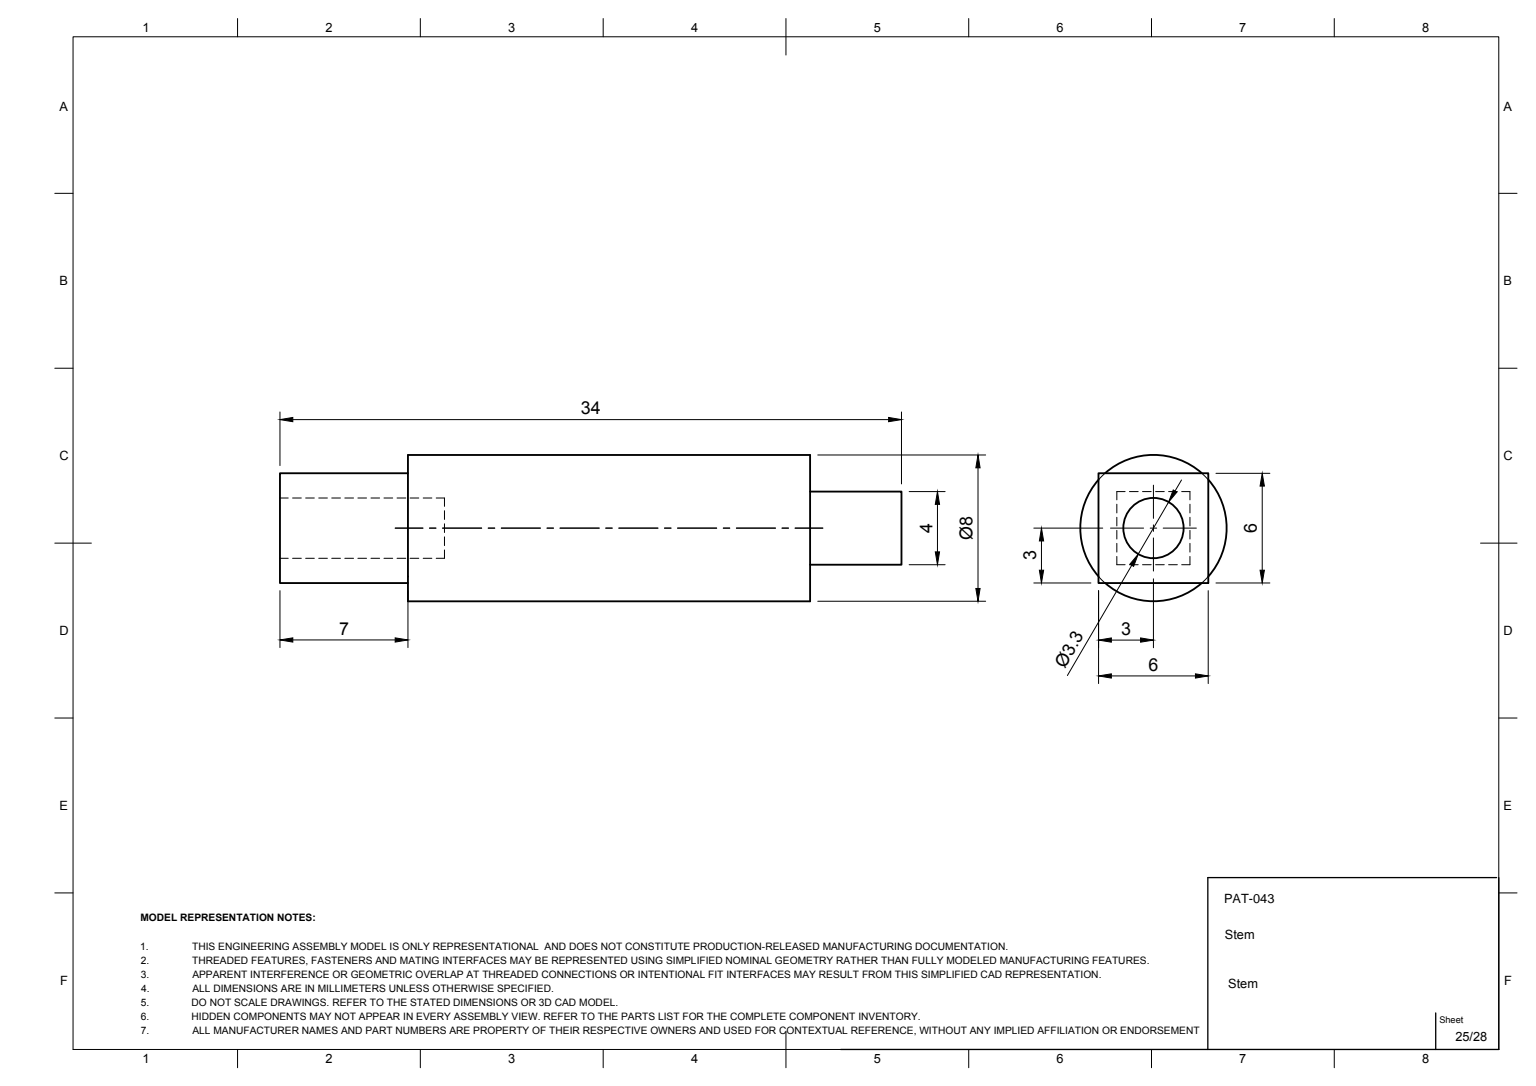
ISO-10303-21;
HEADER;
/* Generated by software containing ST-Developer
 * from STEP Tools, Inc. (www.steptools.com) 
 */

FILE_DESCRIPTION(
/* description */ ('Four-valve pipe header'),
/* implementation_level */ '2;1');

FILE_NAME(
/* name */ 'Stem.step',
/* time_stamp */ '2026-10-29T16:56:19-07:00',
/* author */ (''),
/* organization */ (''),
/* preprocessor_version */ 'ST-DEVELOPER v20.2',
/* originating_system */ 'Autodesk Translation Framework v15.17.0.0',
/* authorisation */ '');

FILE_SCHEMA (('AUTOMOTIVE_DESIGN { 1 0 10303 214 3 1 1 }'));
ENDSEC;

DATA;
#10=MECHANICAL_DESIGN_GEOMETRIC_PRESENTATION_REPRESENTATION('',(#354),#10119);
#302=SHAPE_REPRESENTATION_RELATIONSHIP('SRR','None',#10265,#328);
#328=ADVANCED_BREP_SHAPE_REPRESENTATION('',(#378),#10114);
#354=STYLED_ITEM('',(#10463),#378);
#378=MANIFOLD_SOLID_BREP('Body1',#5602);
#528=FACE_BOUND('',#1466,.T.);
#529=FACE_BOUND('',#1478,.T.);
#698=PLANE('',#6431);
#699=PLANE('',#6432);
#700=PLANE('',#6434);
#701=PLANE('',#6436);
#702=PLANE('',#6438);
#703=PLANE('',#6440);
#704=PLANE('',#6441);
#705=PLANE('',#6442);
#706=PLANE('',#6443);
#707=PLANE('',#6444);
#708=PLANE('',#6445);
#709=PLANE('',#6447);
#710=PLANE('',#6450);
#711=PLANE('',#6452);
#712=PLANE('',#6454);
#713=PLANE('',#6455);
#714=PLANE('',#6456);
#715=PLANE('',#6457);
#716=PLANE('',#6458);
#717=PLANE('',#6461);
#1021=FACE_OUTER_BOUND('',#1455,.T.);
#1022=FACE_OUTER_BOUND('',#1456,.T.);
#1023=FACE_OUTER_BOUND('',#1457,.T.);
#1024=FACE_OUTER_BOUND('',#1458,.T.);
#1025=FACE_OUTER_BOUND('',#1459,.T.);
#1026=FACE_OUTER_BOUND('',#1460,.T.);
#1027=FACE_OUTER_BOUND('',#1461,.T.);
#1028=FACE_OUTER_BOUND('',#1462,.T.);
#1029=FACE_OUTER_BOUND('',#1463,.T.);
#1030=FACE_OUTER_BOUND('',#1464,.T.);
#1031=FACE_OUTER_BOUND('',#1465,.T.);
#1032=FACE_OUTER_BOUND('',#1467,.T.);
#1033=FACE_OUTER_BOUND('',#1468,.T.);
#1034=FACE_OUTER_BOUND('',#1469,.T.);
#1035=FACE_OUTER_BOUND('',#1470,.T.);
#1036=FACE_OUTER_BOUND('',#1471,.T.);
#1037=FACE_OUTER_BOUND('',#1472,.T.);
#1038=FACE_OUTER_BOUND('',#1473,.T.);
#1039=FACE_OUTER_BOUND('',#1474,.T.);
#1040=FACE_OUTER_BOUND('',#1475,.T.);
#1041=FACE_OUTER_BOUND('',#1476,.T.);
#1042=FACE_OUTER_BOUND('',#1477,.T.);
#1455=EDGE_LOOP('',(#4913,#4914,#4915,#4916));
#1456=EDGE_LOOP('',(#4917));
#1457=EDGE_LOOP('',(#4918,#4919,#4920));
#1458=EDGE_LOOP('',(#4921,#4922,#4923));
#1459=EDGE_LOOP('',(#4924,#4925,#4926));
#1460=EDGE_LOOP('',(#4927,#4928,#4929));
#1461=EDGE_LOOP('',(#4930,#4931,#4932,#4933,#4934,#4935));
#1462=EDGE_LOOP('',(#4936,#4937,#4938,#4939,#4940,#4941));
#1463=EDGE_LOOP('',(#4942,#4943,#4944,#4945,#4946,#4947));
#1464=EDGE_LOOP('',(#4948,#4949,#4950,#4951,#4952,#4953));
#1465=EDGE_LOOP('',(#4954,#4955,#4956,#4957));
#1466=EDGE_LOOP('',(#4958));
#1467=EDGE_LOOP('',(#4959,#4960));
#1468=EDGE_LOOP('',(#4961,#4962,#4963));
#1469=EDGE_LOOP('',(#4964,#4965));
#1470=EDGE_LOOP('',(#4966,#4967));
#1471=EDGE_LOOP('',(#4968,#4969,#4970,#4971));
#1472=EDGE_LOOP('',(#4972,#4973,#4974,#4975));
#1473=EDGE_LOOP('',(#4976,#4977,#4978,#4979));
#1474=EDGE_LOOP('',(#4980,#4981,#4982,#4983));
#1475=EDGE_LOOP('',(#4984,#4985,#4986,#4987));
#1476=EDGE_LOOP('',(#4988,#4989,#4990,#4991,#4992,#4993,#4994,#4995,#4996,
#4997,#4998,#4999));
#1477=EDGE_LOOP('',(#5000));
#1478=EDGE_LOOP('',(#5001,#5002,#5003,#5004));
#1843=LINE('',#9751,#2261);
#1844=LINE('',#9759,#2262);
#1845=LINE('',#9760,#2263);
#1846=LINE('',#9766,#2264);
#1847=LINE('',#9767,#2265);
#1848=LINE('',#9773,#2266);
#1849=LINE('',#9774,#2267);
#1850=LINE('',#9780,#2268);
#1851=LINE('',#9781,#2269);
#1852=LINE('',#9783,#2270);
#1853=LINE('',#9785,#2271);
#1854=LINE('',#9787,#2272);
#1855=LINE('',#9788,#2273);
#1856=LINE('',#9790,#2274);
#1857=LINE('',#9792,#2275);
#1858=LINE('',#9793,#2276);
#1859=LINE('',#9795,#2277);
#1860=LINE('',#9797,#2278);
#1861=LINE('',#9798,#2279);
#1862=LINE('',#9800,#2280);
#1863=LINE('',#9801,#2281);
#1864=LINE('',#9816,#2282);
#1865=LINE('',#9818,#2283);
#1866=LINE('',#9820,#2284);
#1867=LINE('',#9821,#2285);
#1868=LINE('',#9824,#2286);
#1869=LINE('',#9826,#2287);
#1870=LINE('',#9827,#2288);
#1871=LINE('',#9830,#2289);
#1872=LINE('',#9832,#2290);
#1873=LINE('',#9833,#2291);
#1874=LINE('',#9835,#2292);
#1875=LINE('',#9836,#2293);
#1876=LINE('',#9840,#2294);
#2261=VECTOR('',#7962,0.165);
#2262=VECTOR('',#7971,1.);
#2263=VECTOR('',#7972,1.);
#2264=VECTOR('',#7977,1.);
#2265=VECTOR('',#7978,1.);
#2266=VECTOR('',#7983,1.);
#2267=VECTOR('',#7984,1.);
#2268=VECTOR('',#7989,1.);
#2269=VECTOR('',#7990,1.);
#2270=VECTOR('',#7993,1.);
#2271=VECTOR('',#7994,1.);
#2272=VECTOR('',#7995,1.);
#2273=VECTOR('',#7996,1.);
#2274=VECTOR('',#7999,1.);
#2275=VECTOR('',#8000,1.);
#2276=VECTOR('',#8001,1.);
#2277=VECTOR('',#8004,1.);
#2278=VECTOR('',#8005,1.);
#2279=VECTOR('',#8006,1.);
#2280=VECTOR('',#8009,1.);
#2281=VECTOR('',#8010,1.);
#2282=VECTOR('',#8033,1.);
#2283=VECTOR('',#8034,1.);
#2284=VECTOR('',#8035,1.);
#2285=VECTOR('',#8036,1.);
#2286=VECTOR('',#8039,1.);
#2287=VECTOR('',#8040,1.);
#2288=VECTOR('',#8041,1.);
#2289=VECTOR('',#8044,1.);
#2290=VECTOR('',#8045,1.);
#2291=VECTOR('',#8046,1.);
#2292=VECTOR('',#8049,1.);
#2293=VECTOR('',#8050,1.);
#2294=VECTOR('',#8055,0.4);
#2557=CIRCLE('',#6429,0.165);
#2558=CIRCLE('',#6430,0.165);
#2559=CIRCLE('',#6433,0.4);
#2560=CIRCLE('',#6435,0.4);
#2561=CIRCLE('',#6437,0.4);
#2562=CIRCLE('',#6439,0.4);
#2563=CIRCLE('',#6446,0.4);
#2564=CIRCLE('',#6448,0.4);
#2565=CIRCLE('',#6449,0.4);
#2566=CIRCLE('',#6451,0.4);
#2567=CIRCLE('',#6453,0.4);
#2568=CIRCLE('',#6460,0.4);
#2962=VERTEX_POINT('',#9748);
#2963=VERTEX_POINT('',#9750);
#2964=VERTEX_POINT('',#9755);
#2965=VERTEX_POINT('',#9756);
#2966=VERTEX_POINT('',#9758);
#2967=VERTEX_POINT('',#9762);
#2968=VERTEX_POINT('',#9763);
#2969=VERTEX_POINT('',#9765);
#2970=VERTEX_POINT('',#9769);
#2971=VERTEX_POINT('',#9770);
#2972=VERTEX_POINT('',#9772);
#2973=VERTEX_POINT('',#9776);
#2974=VERTEX_POINT('',#9777);
#2975=VERTEX_POINT('',#9779);
#2976=VERTEX_POINT('',#9784);
#2977=VERTEX_POINT('',#9786);
#2978=VERTEX_POINT('',#9791);
#2979=VERTEX_POINT('',#9796);
#2980=VERTEX_POINT('',#9806);
#2981=VERTEX_POINT('',#9814);
#2982=VERTEX_POINT('',#9815);
#2983=VERTEX_POINT('',#9817);
#2984=VERTEX_POINT('',#9819);
#2985=VERTEX_POINT('',#9823);
#2986=VERTEX_POINT('',#9825);
#2987=VERTEX_POINT('',#9829);
#2988=VERTEX_POINT('',#9831);
#2989=VERTEX_POINT('',#9839);
#3623=EDGE_CURVE('',#2962,#2962,#2557,.T.);
#3624=EDGE_CURVE('',#2962,#2963,#1843,.T.);
#3625=EDGE_CURVE('',#2963,#2963,#2558,.T.);
#3626=EDGE_CURVE('',#2964,#2965,#2559,.T.);
#3627=EDGE_CURVE('',#2966,#2965,#1844,.T.);
#3628=EDGE_CURVE('',#2964,#2966,#1845,.T.);
#3629=EDGE_CURVE('',#2967,#2968,#2560,.T.);
#3630=EDGE_CURVE('',#2969,#2968,#1846,.T.);
#3631=EDGE_CURVE('',#2967,#2969,#1847,.T.);
#3632=EDGE_CURVE('',#2970,#2971,#2561,.T.);
#3633=EDGE_CURVE('',#2972,#2971,#1848,.T.);
#3634=EDGE_CURVE('',#2970,#2972,#1849,.T.);
#3635=EDGE_CURVE('',#2973,#2974,#2562,.T.);
#3636=EDGE_CURVE('',#2975,#2974,#1850,.T.);
#3637=EDGE_CURVE('',#2973,#2975,#1851,.T.);
#3638=EDGE_CURVE('',#2964,#2974,#1852,.T.);
#3639=EDGE_CURVE('',#2966,#2976,#1853,.T.);
#3640=EDGE_CURVE('',#2977,#2976,#1854,.T.);
#3641=EDGE_CURVE('',#2975,#2977,#1855,.T.);
#3642=EDGE_CURVE('',#2973,#2971,#1856,.T.);
#3643=EDGE_CURVE('',#2978,#2977,#1857,.T.);
#3644=EDGE_CURVE('',#2972,#2978,#1858,.T.);
#3645=EDGE_CURVE('',#2970,#2968,#1859,.T.);
#3646=EDGE_CURVE('',#2979,#2978,#1860,.T.);
#3647=EDGE_CURVE('',#2969,#2979,#1861,.T.);
#3648=EDGE_CURVE('',#2967,#2965,#1862,.T.);
#3649=EDGE_CURVE('',#2976,#2979,#1863,.T.);
#3650=EDGE_CURVE('',#2968,#2970,#2563,.T.);
#3651=EDGE_CURVE('',#2965,#2980,#2564,.T.);
#3652=EDGE_CURVE('',#2980,#2967,#2565,.T.);
#3653=EDGE_CURVE('',#2974,#2964,#2566,.T.);
#3654=EDGE_CURVE('',#2971,#2973,#2567,.T.);
#3655=EDGE_CURVE('',#2981,#2982,#1864,.T.);
#3656=EDGE_CURVE('',#2982,#2983,#1865,.T.);
#3657=EDGE_CURVE('',#2984,#2983,#1866,.T.);
#3658=EDGE_CURVE('',#2981,#2984,#1867,.T.);
#3659=EDGE_CURVE('',#2985,#2981,#1868,.T.);
#3660=EDGE_CURVE('',#2986,#2984,#1869,.T.);
#3661=EDGE_CURVE('',#2985,#2986,#1870,.T.);
#3662=EDGE_CURVE('',#2987,#2985,#1871,.T.);
#3663=EDGE_CURVE('',#2988,#2986,#1872,.T.);
#3664=EDGE_CURVE('',#2987,#2988,#1873,.T.);
#3665=EDGE_CURVE('',#2982,#2987,#1874,.T.);
#3666=EDGE_CURVE('',#2983,#2988,#1875,.T.);
#3667=EDGE_CURVE('',#2980,#2989,#1876,.T.);
#3668=EDGE_CURVE('',#2989,#2989,#2568,.T.);
#4913=ORIENTED_EDGE('',*,*,#3623,.F.);
#4914=ORIENTED_EDGE('',*,*,#3624,.T.);
#4915=ORIENTED_EDGE('',*,*,#3625,.F.);
#4916=ORIENTED_EDGE('',*,*,#3624,.F.);
#4917=ORIENTED_EDGE('',*,*,#3623,.T.);
#4918=ORIENTED_EDGE('',*,*,#3626,.T.);
#4919=ORIENTED_EDGE('',*,*,#3627,.F.);
#4920=ORIENTED_EDGE('',*,*,#3628,.F.);
#4921=ORIENTED_EDGE('',*,*,#3629,.T.);
#4922=ORIENTED_EDGE('',*,*,#3630,.F.);
#4923=ORIENTED_EDGE('',*,*,#3631,.F.);
#4924=ORIENTED_EDGE('',*,*,#3632,.T.);
#4925=ORIENTED_EDGE('',*,*,#3633,.F.);
#4926=ORIENTED_EDGE('',*,*,#3634,.F.);
#4927=ORIENTED_EDGE('',*,*,#3635,.T.);
#4928=ORIENTED_EDGE('',*,*,#3636,.F.);
#4929=ORIENTED_EDGE('',*,*,#3637,.F.);
#4930=ORIENTED_EDGE('',*,*,#3636,.T.);
#4931=ORIENTED_EDGE('',*,*,#3638,.F.);
#4932=ORIENTED_EDGE('',*,*,#3628,.T.);
#4933=ORIENTED_EDGE('',*,*,#3639,.T.);
#4934=ORIENTED_EDGE('',*,*,#3640,.F.);
#4935=ORIENTED_EDGE('',*,*,#3641,.F.);
#4936=ORIENTED_EDGE('',*,*,#3633,.T.);
#4937=ORIENTED_EDGE('',*,*,#3642,.F.);
#4938=ORIENTED_EDGE('',*,*,#3637,.T.);
#4939=ORIENTED_EDGE('',*,*,#3641,.T.);
#4940=ORIENTED_EDGE('',*,*,#3643,.F.);
#4941=ORIENTED_EDGE('',*,*,#3644,.F.);
#4942=ORIENTED_EDGE('',*,*,#3630,.T.);
#4943=ORIENTED_EDGE('',*,*,#3645,.F.);
#4944=ORIENTED_EDGE('',*,*,#3634,.T.);
#4945=ORIENTED_EDGE('',*,*,#3644,.T.);
#4946=ORIENTED_EDGE('',*,*,#3646,.F.);
#4947=ORIENTED_EDGE('',*,*,#3647,.F.);
#4948=ORIENTED_EDGE('',*,*,#3627,.T.);
#4949=ORIENTED_EDGE('',*,*,#3648,.F.);
#4950=ORIENTED_EDGE('',*,*,#3631,.T.);
#4951=ORIENTED_EDGE('',*,*,#3647,.T.);
#4952=ORIENTED_EDGE('',*,*,#3649,.F.);
#4953=ORIENTED_EDGE('',*,*,#3639,.F.);
#4954=ORIENTED_EDGE('',*,*,#3649,.T.);
#4955=ORIENTED_EDGE('',*,*,#3646,.T.);
#4956=ORIENTED_EDGE('',*,*,#3643,.T.);
#4957=ORIENTED_EDGE('',*,*,#3640,.T.);
#4958=ORIENTED_EDGE('',*,*,#3625,.T.);
#4959=ORIENTED_EDGE('',*,*,#3645,.T.);
#4960=ORIENTED_EDGE('',*,*,#3650,.T.);
#4961=ORIENTED_EDGE('',*,*,#3648,.T.);
#4962=ORIENTED_EDGE('',*,*,#3651,.T.);
#4963=ORIENTED_EDGE('',*,*,#3652,.T.);
#4964=ORIENTED_EDGE('',*,*,#3638,.T.);
#4965=ORIENTED_EDGE('',*,*,#3653,.T.);
#4966=ORIENTED_EDGE('',*,*,#3642,.T.);
#4967=ORIENTED_EDGE('',*,*,#3654,.T.);
#4968=ORIENTED_EDGE('',*,*,#3655,.T.);
#4969=ORIENTED_EDGE('',*,*,#3656,.T.);
#4970=ORIENTED_EDGE('',*,*,#3657,.F.);
#4971=ORIENTED_EDGE('',*,*,#3658,.F.);
#4972=ORIENTED_EDGE('',*,*,#3659,.T.);
#4973=ORIENTED_EDGE('',*,*,#3658,.T.);
#4974=ORIENTED_EDGE('',*,*,#3660,.F.);
#4975=ORIENTED_EDGE('',*,*,#3661,.F.);
#4976=ORIENTED_EDGE('',*,*,#3662,.T.);
#4977=ORIENTED_EDGE('',*,*,#3661,.T.);
#4978=ORIENTED_EDGE('',*,*,#3663,.F.);
#4979=ORIENTED_EDGE('',*,*,#3664,.F.);
#4980=ORIENTED_EDGE('',*,*,#3665,.T.);
#4981=ORIENTED_EDGE('',*,*,#3664,.T.);
#4982=ORIENTED_EDGE('',*,*,#3666,.F.);
#4983=ORIENTED_EDGE('',*,*,#3656,.F.);
#4984=ORIENTED_EDGE('',*,*,#3665,.F.);
#4985=ORIENTED_EDGE('',*,*,#3655,.F.);
#4986=ORIENTED_EDGE('',*,*,#3659,.F.);
#4987=ORIENTED_EDGE('',*,*,#3662,.F.);
#4988=ORIENTED_EDGE('',*,*,#3651,.F.);
#4989=ORIENTED_EDGE('',*,*,#3626,.F.);
#4990=ORIENTED_EDGE('',*,*,#3653,.F.);
#4991=ORIENTED_EDGE('',*,*,#3635,.F.);
#4992=ORIENTED_EDGE('',*,*,#3654,.F.);
#4993=ORIENTED_EDGE('',*,*,#3632,.F.);
#4994=ORIENTED_EDGE('',*,*,#3650,.F.);
#4995=ORIENTED_EDGE('',*,*,#3629,.F.);
#4996=ORIENTED_EDGE('',*,*,#3652,.F.);
#4997=ORIENTED_EDGE('',*,*,#3667,.T.);
#4998=ORIENTED_EDGE('',*,*,#3668,.T.);
#4999=ORIENTED_EDGE('',*,*,#3667,.F.);
#5000=ORIENTED_EDGE('',*,*,#3668,.F.);
#5001=ORIENTED_EDGE('',*,*,#3657,.T.);
#5002=ORIENTED_EDGE('',*,*,#3666,.T.);
#5003=ORIENTED_EDGE('',*,*,#3663,.T.);
#5004=ORIENTED_EDGE('',*,*,#3660,.T.);
#5241=CYLINDRICAL_SURFACE('',#6428,0.165);
#5242=CYLINDRICAL_SURFACE('',#6459,0.4);
#5521=ADVANCED_FACE('',(#1021),#5241,.F.);
#5522=ADVANCED_FACE('',(#1022),#698,.T.);
#5523=ADVANCED_FACE('',(#1023),#699,.F.);
#5524=ADVANCED_FACE('',(#1024),#700,.F.);
#5525=ADVANCED_FACE('',(#1025),#701,.F.);
#5526=ADVANCED_FACE('',(#1026),#702,.F.);
#5527=ADVANCED_FACE('',(#1027),#703,.T.);
#5528=ADVANCED_FACE('',(#1028),#704,.T.);
#5529=ADVANCED_FACE('',(#1029),#705,.T.);
#5530=ADVANCED_FACE('',(#1030),#706,.T.);
#5531=ADVANCED_FACE('',(#1031,#528),#707,.T.);
#5532=ADVANCED_FACE('',(#1032),#708,.T.);
#5533=ADVANCED_FACE('',(#1033),#709,.T.);
#5534=ADVANCED_FACE('',(#1034),#710,.T.);
#5535=ADVANCED_FACE('',(#1035),#711,.T.);
#5536=ADVANCED_FACE('',(#1036),#712,.T.);
#5537=ADVANCED_FACE('',(#1037),#713,.T.);
#5538=ADVANCED_FACE('',(#1038),#714,.T.);
#5539=ADVANCED_FACE('',(#1039),#715,.T.);
#5540=ADVANCED_FACE('',(#1040),#716,.F.);
#5541=ADVANCED_FACE('',(#1041),#5242,.T.);
#5542=ADVANCED_FACE('',(#1042,#529),#717,.F.);
#5602=CLOSED_SHELL('',(#5521,#5522,#5523,#5524,#5525,#5526,#5527,#5528,
#5529,#5530,#5531,#5532,#5533,#5534,#5535,#5536,#5537,#5538,#5539,#5540,
#5541,#5542));
#6427=AXIS2_PLACEMENT_3D('',#9746,#7956,#7957);
#6428=AXIS2_PLACEMENT_3D('',#9747,#7958,#7959);
#6429=AXIS2_PLACEMENT_3D('',#9749,#7960,#7961);
#6430=AXIS2_PLACEMENT_3D('',#9752,#7963,#7964);
#6431=AXIS2_PLACEMENT_3D('',#9753,#7965,#7966);
#6432=AXIS2_PLACEMENT_3D('',#9754,#7967,#7968);
#6433=AXIS2_PLACEMENT_3D('',#9757,#7969,#7970);
#6434=AXIS2_PLACEMENT_3D('',#9761,#7973,#7974);
#6435=AXIS2_PLACEMENT_3D('',#9764,#7975,#7976);
#6436=AXIS2_PLACEMENT_3D('',#9768,#7979,#7980);
#6437=AXIS2_PLACEMENT_3D('',#9771,#7981,#7982);
#6438=AXIS2_PLACEMENT_3D('',#9775,#7985,#7986);
#6439=AXIS2_PLACEMENT_3D('',#9778,#7987,#7988);
#6440=AXIS2_PLACEMENT_3D('',#9782,#7991,#7992);
#6441=AXIS2_PLACEMENT_3D('',#9789,#7997,#7998);
#6442=AXIS2_PLACEMENT_3D('',#9794,#8002,#8003);
#6443=AXIS2_PLACEMENT_3D('',#9799,#8007,#8008);
#6444=AXIS2_PLACEMENT_3D('',#9802,#8011,#8012);
#6445=AXIS2_PLACEMENT_3D('',#9803,#8013,#8014);
#6446=AXIS2_PLACEMENT_3D('',#9804,#8015,#8016);
#6447=AXIS2_PLACEMENT_3D('',#9805,#8017,#8018);
#6448=AXIS2_PLACEMENT_3D('',#9807,#8019,#8020);
#6449=AXIS2_PLACEMENT_3D('',#9808,#8021,#8022);
#6450=AXIS2_PLACEMENT_3D('',#9809,#8023,#8024);
#6451=AXIS2_PLACEMENT_3D('',#9810,#8025,#8026);
#6452=AXIS2_PLACEMENT_3D('',#9811,#8027,#8028);
#6453=AXIS2_PLACEMENT_3D('',#9812,#8029,#8030);
#6454=AXIS2_PLACEMENT_3D('',#9813,#8031,#8032);
#6455=AXIS2_PLACEMENT_3D('',#9822,#8037,#8038);
#6456=AXIS2_PLACEMENT_3D('',#9828,#8042,#8043);
#6457=AXIS2_PLACEMENT_3D('',#9834,#8047,#8048);
#6458=AXIS2_PLACEMENT_3D('',#9837,#8051,#8052);
#6459=AXIS2_PLACEMENT_3D('',#9838,#8053,#8054);
#6460=AXIS2_PLACEMENT_3D('',#9841,#8056,#8057);
#6461=AXIS2_PLACEMENT_3D('',#9842,#8058,#8059);
#7956=DIRECTION('axis',(0.,0.,1.));
#7957=DIRECTION('refdir',(1.,0.,0.));
#7958=DIRECTION('center_axis',(0.,0.,1.));
#7959=DIRECTION('ref_axis',(1.,0.,0.));
#7960=DIRECTION('center_axis',(0.,0.,1.));
#7961=DIRECTION('ref_axis',(1.,0.,0.));
#7962=DIRECTION('',(0.,0.,1.));
#7963=DIRECTION('center_axis',(0.,0.,-1.));
#7964=DIRECTION('ref_axis',(1.,0.,0.));
#7965=DIRECTION('center_axis',(0.,0.,1.));
#7966=DIRECTION('ref_axis',(1.,0.,0.));
#7967=DIRECTION('center_axis',(0.,0.,1.));
#7968=DIRECTION('ref_axis',(1.,0.,0.));
#7969=DIRECTION('center_axis',(0.,0.,1.));
#7970=DIRECTION('ref_axis',(1.,0.,0.));
#7971=DIRECTION('',(0.,-1.,0.));
#7972=DIRECTION('',(-1.,0.,0.));
#7973=DIRECTION('center_axis',(0.,0.,1.));
#7974=DIRECTION('ref_axis',(1.,0.,0.));
#7975=DIRECTION('center_axis',(0.,0.,1.));
#7976=DIRECTION('ref_axis',(1.,0.,0.));
#7977=DIRECTION('',(1.,0.,0.));
#7978=DIRECTION('',(0.,-1.,0.));
#7979=DIRECTION('center_axis',(0.,0.,1.));
#7980=DIRECTION('ref_axis',(1.,0.,0.));
#7981=DIRECTION('center_axis',(0.,0.,1.));
#7982=DIRECTION('ref_axis',(1.,0.,0.));
#7983=DIRECTION('',(0.,1.,0.));
#7984=DIRECTION('',(1.,0.,0.));
#7985=DIRECTION('center_axis',(0.,0.,1.));
#7986=DIRECTION('ref_axis',(1.,0.,0.));
#7987=DIRECTION('center_axis',(0.,0.,1.));
#7988=DIRECTION('ref_axis',(1.,0.,0.));
#7989=DIRECTION('',(-1.,0.,0.));
#7990=DIRECTION('',(0.,1.,0.));
#7991=DIRECTION('center_axis',(0.,1.,0.));
#7992=DIRECTION('ref_axis',(-1.,0.,0.));
#7993=DIRECTION('',(1.,0.,0.));
#7994=DIRECTION('',(0.,0.,1.));
#7995=DIRECTION('',(-1.,0.,0.));
#7996=DIRECTION('',(0.,0.,1.));
#7997=DIRECTION('center_axis',(1.,0.,0.));
#7998=DIRECTION('ref_axis',(0.,1.,0.));
#7999=DIRECTION('',(0.,-1.,0.));
#8000=DIRECTION('',(0.,1.,0.));
#8001=DIRECTION('',(0.,0.,1.));
#8002=DIRECTION('center_axis',(0.,-1.,0.));
#8003=DIRECTION('ref_axis',(1.,0.,0.));
#8004=DIRECTION('',(-1.,0.,0.));
#8005=DIRECTION('',(1.,0.,0.));
#8006=DIRECTION('',(0.,0.,1.));
#8007=DIRECTION('center_axis',(-1.,0.,0.));
#8008=DIRECTION('ref_axis',(0.,-1.,0.));
#8009=DIRECTION('',(0.,1.,0.));
#8010=DIRECTION('',(0.,-1.,0.));
#8011=DIRECTION('center_axis',(0.,0.,1.));
#8012=DIRECTION('ref_axis',(1.,0.,0.));
#8013=DIRECTION('center_axis',(0.,0.,1.));
#8014=DIRECTION('ref_axis',(1.,0.,0.));
#8015=DIRECTION('center_axis',(0.,0.,1.));
#8016=DIRECTION('ref_axis',(1.,0.,0.));
#8017=DIRECTION('center_axis',(0.,0.,1.));
#8018=DIRECTION('ref_axis',(1.,0.,0.));
#8019=DIRECTION('center_axis',(0.,0.,1.));
#8020=DIRECTION('ref_axis',(1.,0.,0.));
#8021=DIRECTION('center_axis',(0.,0.,1.));
#8022=DIRECTION('ref_axis',(1.,0.,0.));
#8023=DIRECTION('center_axis',(0.,0.,1.));
#8024=DIRECTION('ref_axis',(1.,0.,0.));
#8025=DIRECTION('center_axis',(0.,0.,1.));
#8026=DIRECTION('ref_axis',(1.,0.,0.));
#8027=DIRECTION('center_axis',(0.,0.,1.));
#8028=DIRECTION('ref_axis',(1.,0.,0.));
#8029=DIRECTION('center_axis',(0.,0.,1.));
#8030=DIRECTION('ref_axis',(1.,0.,0.));
#8031=DIRECTION('center_axis',(0.,1.,0.));
#8032=DIRECTION('ref_axis',(-1.,0.,0.));
#8033=DIRECTION('',(-1.,0.,0.));
#8034=DIRECTION('',(0.,0.,1.));
#8035=DIRECTION('',(-1.,0.,0.));
#8036=DIRECTION('',(0.,0.,1.));
#8037=DIRECTION('center_axis',(1.,0.,0.));
#8038=DIRECTION('ref_axis',(0.,1.,0.));
#8039=DIRECTION('',(0.,1.,0.));
#8040=DIRECTION('',(0.,1.,0.));
#8041=DIRECTION('',(0.,0.,1.));
#8042=DIRECTION('center_axis',(0.,-1.,0.));
#8043=DIRECTION('ref_axis',(1.,0.,0.));
#8044=DIRECTION('',(1.,0.,0.));
#8045=DIRECTION('',(1.,0.,0.));
#8046=DIRECTION('',(0.,0.,1.));
#8047=DIRECTION('center_axis',(-1.,0.,0.));
#8048=DIRECTION('ref_axis',(0.,-1.,0.));
#8049=DIRECTION('',(0.,-1.,0.));
#8050=DIRECTION('',(0.,-1.,0.));
#8051=DIRECTION('center_axis',(0.,0.,1.));
#8052=DIRECTION('ref_axis',(1.,0.,0.));
#8053=DIRECTION('center_axis',(0.,0.,1.));
#8054=DIRECTION('ref_axis',(1.,0.,0.));
#8055=DIRECTION('',(0.,0.,-1.));
#8056=DIRECTION('center_axis',(0.,0.,1.));
#8057=DIRECTION('ref_axis',(1.,0.,0.));
#8058=DIRECTION('center_axis',(0.,0.,1.));
#8059=DIRECTION('ref_axis',(1.,0.,0.));
#9746=CARTESIAN_POINT('',(0.,0.,0.));
#9747=CARTESIAN_POINT('Origin',(0.,0.,8.5));
#9748=CARTESIAN_POINT('',(-0.165,-2.02066721859313E-17,8.5));
#9749=CARTESIAN_POINT('Origin',(0.,0.,8.5));
#9750=CARTESIAN_POINT('',(-0.165,2.02066721859313E-17,9.4));
#9751=CARTESIAN_POINT('',(-0.165,-2.02066721859313E-17,8.5));
#9752=CARTESIAN_POINT('Origin',(0.,0.,9.4));
#9753=CARTESIAN_POINT('Origin',(0.,0.,8.5));
#9754=CARTESIAN_POINT('Origin',(0.,0.,8.7));
#9755=CARTESIAN_POINT('',(-0.264575131106459,0.3,8.7));
#9756=CARTESIAN_POINT('',(-0.3,0.264575131106459,8.7));
#9757=CARTESIAN_POINT('Origin',(0.,0.,8.7));
#9758=CARTESIAN_POINT('',(-0.3,0.3,8.7));
#9759=CARTESIAN_POINT('',(-0.3,0.3,8.7));
#9760=CARTESIAN_POINT('',(0.3,0.3,8.7));
#9761=CARTESIAN_POINT('Origin',(0.,0.,8.7));
#9762=CARTESIAN_POINT('',(-0.3,-0.264575131106459,8.7));
#9763=CARTESIAN_POINT('',(-0.264575131106459,-0.3,8.7));
#9764=CARTESIAN_POINT('Origin',(0.,0.,8.7));
#9765=CARTESIAN_POINT('',(-0.3,-0.3,8.7));
#9766=CARTESIAN_POINT('',(-0.3,-0.3,8.7));
#9767=CARTESIAN_POINT('',(-0.3,0.3,8.7));
#9768=CARTESIAN_POINT('Origin',(0.,0.,8.7));
#9769=CARTESIAN_POINT('',(0.264575131106459,-0.3,8.7));
#9770=CARTESIAN_POINT('',(0.3,-0.264575131106459,8.7));
#9771=CARTESIAN_POINT('Origin',(0.,0.,8.7));
#9772=CARTESIAN_POINT('',(0.3,-0.3,8.7));
#9773=CARTESIAN_POINT('',(0.3,-0.3,8.7));
#9774=CARTESIAN_POINT('',(-0.3,-0.3,8.7));
#9775=CARTESIAN_POINT('Origin',(0.,0.,8.7));
#9776=CARTESIAN_POINT('',(0.3,0.264575131106459,8.7));
#9777=CARTESIAN_POINT('',(0.264575131106459,0.3,8.7));
#9778=CARTESIAN_POINT('Origin',(0.,0.,8.7));
#9779=CARTESIAN_POINT('',(0.3,0.3,8.7));
#9780=CARTESIAN_POINT('',(0.3,0.3,8.7));
#9781=CARTESIAN_POINT('',(0.3,-0.3,8.7));
#9782=CARTESIAN_POINT('Origin',(0.3,0.3,8.7));
#9783=CARTESIAN_POINT('',(0.15,0.3,8.7));
#9784=CARTESIAN_POINT('',(-0.3,0.3,9.4));
#9785=CARTESIAN_POINT('',(-0.3,0.3,8.7));
#9786=CARTESIAN_POINT('',(0.3,0.3,9.4));
#9787=CARTESIAN_POINT('',(0.3,0.3,9.4));
#9788=CARTESIAN_POINT('',(0.3,0.3,8.7));
#9789=CARTESIAN_POINT('Origin',(0.3,-0.3,8.7));
#9790=CARTESIAN_POINT('',(0.3,-0.15,8.7));
#9791=CARTESIAN_POINT('',(0.3,-0.3,9.4));
#9792=CARTESIAN_POINT('',(0.3,-0.3,9.4));
#9793=CARTESIAN_POINT('',(0.3,-0.3,8.7));
#9794=CARTESIAN_POINT('Origin',(-0.3,-0.3,8.7));
#9795=CARTESIAN_POINT('',(-0.15,-0.3,8.7));
#9796=CARTESIAN_POINT('',(-0.3,-0.3,9.4));
#9797=CARTESIAN_POINT('',(-0.3,-0.3,9.4));
#9798=CARTESIAN_POINT('',(-0.3,-0.3,8.7));
#9799=CARTESIAN_POINT('Origin',(-0.3,0.3,8.7));
#9800=CARTESIAN_POINT('',(-0.3,0.15,8.7));
#9801=CARTESIAN_POINT('',(-0.3,0.3,9.4));
#9802=CARTESIAN_POINT('Origin',(0.,0.,9.4));
#9803=CARTESIAN_POINT('Origin',(0.,0.,8.7));
#9804=CARTESIAN_POINT('Origin',(0.,0.,8.7));
#9805=CARTESIAN_POINT('Origin',(0.,0.,8.7));
#9806=CARTESIAN_POINT('',(-0.4,-4.89858719658941E-17,8.7));
#9807=CARTESIAN_POINT('Origin',(0.,0.,8.7));
#9808=CARTESIAN_POINT('Origin',(0.,0.,8.7));
#9809=CARTESIAN_POINT('Origin',(0.,0.,8.7));
#9810=CARTESIAN_POINT('Origin',(0.,0.,8.7));
#9811=CARTESIAN_POINT('Origin',(0.,0.,8.7));
#9812=CARTESIAN_POINT('Origin',(0.,0.,8.7));
#9813=CARTESIAN_POINT('Origin',(0.2,0.2,6.));
#9814=CARTESIAN_POINT('',(0.2,0.2,6.));
#9815=CARTESIAN_POINT('',(-0.2,0.2,6.));
#9816=CARTESIAN_POINT('',(0.2,0.2,6.));
#9817=CARTESIAN_POINT('',(-0.2,0.2,6.5));
#9818=CARTESIAN_POINT('',(-0.2,0.2,6.));
#9819=CARTESIAN_POINT('',(0.2,0.2,6.5));
#9820=CARTESIAN_POINT('',(0.1,0.2,6.5));
#9821=CARTESIAN_POINT('',(0.2,0.2,6.));
#9822=CARTESIAN_POINT('Origin',(0.2,-0.2,6.));
#9823=CARTESIAN_POINT('',(0.2,-0.2,6.));
#9824=CARTESIAN_POINT('',(0.2,-0.2,6.));
#9825=CARTESIAN_POINT('',(0.2,-0.2,6.5));
#9826=CARTESIAN_POINT('',(0.2,-0.1,6.5));
#9827=CARTESIAN_POINT('',(0.2,-0.2,6.));
#9828=CARTESIAN_POINT('Origin',(-0.2,-0.2,6.));
#9829=CARTESIAN_POINT('',(-0.2,-0.2,6.));
#9830=CARTESIAN_POINT('',(-0.2,-0.2,6.));
#9831=CARTESIAN_POINT('',(-0.2,-0.2,6.5));
#9832=CARTESIAN_POINT('',(-0.1,-0.2,6.5));
#9833=CARTESIAN_POINT('',(-0.2,-0.2,6.));
#9834=CARTESIAN_POINT('Origin',(-0.2,0.2,6.));
#9835=CARTESIAN_POINT('',(-0.2,0.2,6.));
#9836=CARTESIAN_POINT('',(-0.2,0.1,6.5));
#9837=CARTESIAN_POINT('Origin',(0.,0.,6.));
#9838=CARTESIAN_POINT('Origin',(0.,0.,6.5));
#9839=CARTESIAN_POINT('',(-0.4,-4.89858719658941E-17,6.5));
#9840=CARTESIAN_POINT('',(-0.4,-4.89858719658941E-17,6.5));
#9841=CARTESIAN_POINT('Origin',(0.,0.,6.5));
#9842=CARTESIAN_POINT('Origin',(0.,0.,6.5));
#10083=UNCERTAINTY_MEASURE_WITH_UNIT(LENGTH_MEASURE(0.001),#10120,
'DISTANCE_ACCURACY_VALUE',
'Maximum model space distance between geometric entities at asserted c
onnectivities');
#10088=UNCERTAINTY_MEASURE_WITH_UNIT(LENGTH_MEASURE(0.001),#10120,
'DISTANCE_ACCURACY_VALUE',
'Maximum model space distance between geometric entities at asserted c
onnectivities');
#10114=(
GEOMETRIC_REPRESENTATION_CONTEXT(3)
GLOBAL_UNCERTAINTY_ASSIGNED_CONTEXT((#10083))
GLOBAL_UNIT_ASSIGNED_CONTEXT((#10120,#10122,#10123))
REPRESENTATION_CONTEXT('','3D')
);
#10119=(
GEOMETRIC_REPRESENTATION_CONTEXT(3)
GLOBAL_UNCERTAINTY_ASSIGNED_CONTEXT((#10088))
GLOBAL_UNIT_ASSIGNED_CONTEXT((#10120,#10122,#10123))
REPRESENTATION_CONTEXT('','3D')
);
#10120=(
LENGTH_UNIT()
NAMED_UNIT(*)
SI_UNIT(.CENTI.,.METRE.)
);
#10122=(
NAMED_UNIT(*)
PLANE_ANGLE_UNIT()
SI_UNIT($,.RADIAN.)
);
#10123=(
NAMED_UNIT(*)
SI_UNIT($,.STERADIAN.)
SOLID_ANGLE_UNIT()
);
#10149=SHAPE_DEFINITION_REPRESENTATION(#10179,#10265);
#10179=PRODUCT_DEFINITION_SHAPE('',$,#10296);
#10265=SHAPE_REPRESENTATION('',(#6427),#10114);
#10270=PRODUCT_DEFINITION_CONTEXT('part definition',#10362,'design');
#10296=PRODUCT_DEFINITION('Stem','Stem',#10326,#10270);
#10326=PRODUCT_DEFINITION_FORMATION('',$,#10389);
#10362=APPLICATION_CONTEXT(
'Core Data for Automotive Mechanical Design Process');
#10363=PRODUCT_CONTEXT('part definition',#10362,'mechanical');
#10389=PRODUCT('Stem','Stem','Stem',(#10363));
#10457=COLOUR_RGB('Sky Blue',0.24,0.69,0.87);
#10458=FILL_AREA_STYLE_COLOUR('',#10457);
#10459=FILL_AREA_STYLE('',(#10458));
#10460=SURFACE_STYLE_FILL_AREA(#10459);
#10461=SURFACE_SIDE_STYLE('',(#10460));
#10462=SURFACE_STYLE_USAGE(.BOTH.,#10461);
#10463=PRESENTATION_STYLE_ASSIGNMENT((#10462));
ENDSEC;
END-ISO-10303-21;
